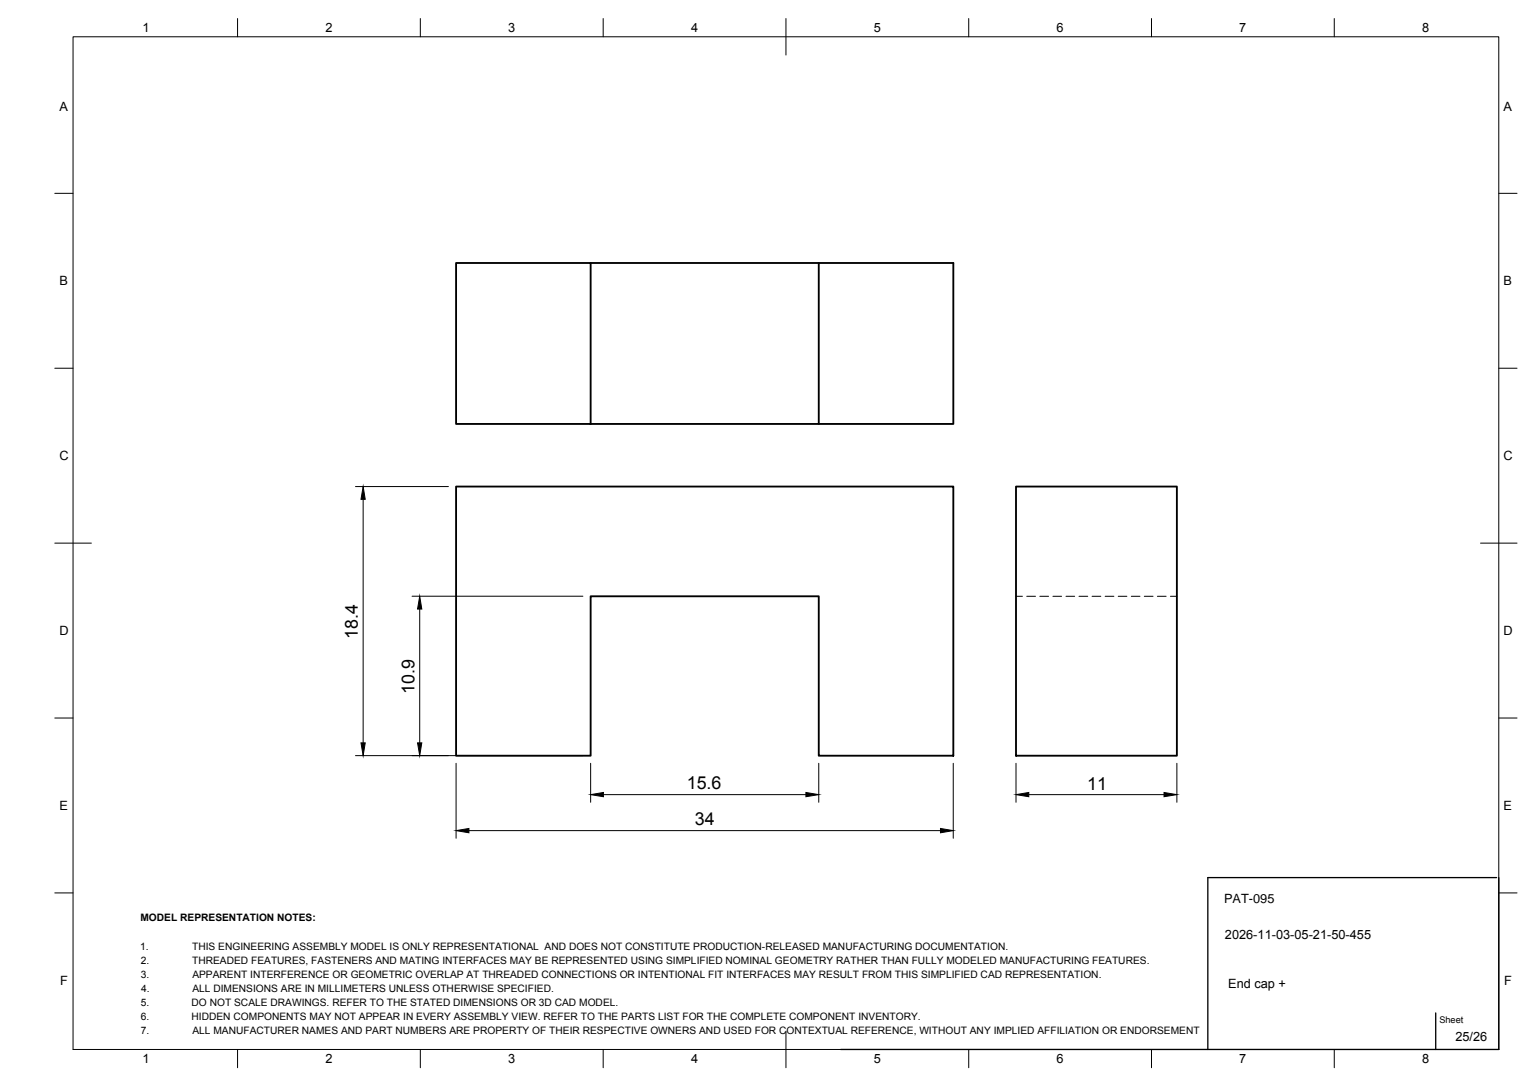
ISO-10303-21;
HEADER;
/* Generated by software containing ST-Developer
 * from STEP Tools, Inc. (www.steptools.com) 
 */

FILE_DESCRIPTION(
/* description */ ('Single-Axis Profile-Rail Linear Slide'),
/* implementation_level */ '2;1');

FILE_NAME(
/* name */ 'End cap +.step',
/* time_stamp */ '2026-10-27T10:47:43-07:00',
/* author */ (''),
/* organization */ (''),
/* preprocessor_version */ 'ST-DEVELOPER v20.2',
/* originating_system */ 'Autodesk Translation Framework v15.17.0.0',
/* authorisation */ '');

FILE_SCHEMA (('AUTOMOTIVE_DESIGN { 1 0 10303 214 3 1 1 }'));
ENDSEC;

DATA;
#10=MECHANICAL_DESIGN_GEOMETRIC_PRESENTATION_REPRESENTATION('',(#348),#14478);
#294=SHAPE_REPRESENTATION_RELATIONSHIP('SRR','None',#14626,#321);
#321=ADVANCED_BREP_SHAPE_REPRESENTATION('',(#373),#14470);
#348=STYLED_ITEM('',(#14824),#373);
#373=MANIFOLD_SOLID_BREP('Body1',#8610);
#781=PLANE('',#9433);
#782=PLANE('',#9434);
#783=PLANE('',#9435);
#784=PLANE('',#9436);
#785=PLANE('',#9437);
#786=PLANE('',#9438);
#787=PLANE('',#9439);
#788=PLANE('',#9440);
#789=PLANE('',#9441);
#790=PLANE('',#9442);
#1210=FACE_OUTER_BOUND('',#1746,.T.);
#1211=FACE_OUTER_BOUND('',#1747,.T.);
#1212=FACE_OUTER_BOUND('',#1748,.T.);
#1213=FACE_OUTER_BOUND('',#1749,.T.);
#1214=FACE_OUTER_BOUND('',#1750,.T.);
#1215=FACE_OUTER_BOUND('',#1751,.T.);
#1216=FACE_OUTER_BOUND('',#1752,.T.);
#1217=FACE_OUTER_BOUND('',#1753,.T.);
#1218=FACE_OUTER_BOUND('',#1754,.T.);
#1219=FACE_OUTER_BOUND('',#1755,.T.);
#1746=EDGE_LOOP('',(#7739,#7740,#7741,#7742));
#1747=EDGE_LOOP('',(#7743,#7744,#7745,#7746));
#1748=EDGE_LOOP('',(#7747,#7748,#7749,#7750));
#1749=EDGE_LOOP('',(#7751,#7752,#7753,#7754));
#1750=EDGE_LOOP('',(#7755,#7756,#7757,#7758));
#1751=EDGE_LOOP('',(#7759,#7760,#7761,#7762));
#1752=EDGE_LOOP('',(#7763,#7764,#7765,#7766));
#1753=EDGE_LOOP('',(#7767,#7768,#7769,#7770));
#1754=EDGE_LOOP('',(#7771,#7772,#7773,#7774,#7775,#7776,#7777,#7778));
#1755=EDGE_LOOP('',(#7779,#7780,#7781,#7782,#7783,#7784,#7785,#7786));
#2683=LINE('',#13996,#3654);
#2684=LINE('',#13998,#3655);
#2685=LINE('',#14000,#3656);
#2686=LINE('',#14001,#3657);
#2687=LINE('',#14004,#3658);
#2688=LINE('',#14006,#3659);
#2689=LINE('',#14007,#3660);
#2690=LINE('',#14010,#3661);
#2691=LINE('',#14012,#3662);
#2692=LINE('',#14013,#3663);
#2693=LINE('',#14016,#3664);
#2694=LINE('',#14018,#3665);
#2695=LINE('',#14019,#3666);
#2696=LINE('',#14022,#3667);
#2697=LINE('',#14024,#3668);
#2698=LINE('',#14025,#3669);
#2699=LINE('',#14028,#3670);
#2700=LINE('',#14030,#3671);
#2701=LINE('',#14031,#3672);
#2702=LINE('',#14034,#3673);
#2703=LINE('',#14036,#3674);
#2704=LINE('',#14037,#3675);
#2705=LINE('',#14039,#3676);
#2706=LINE('',#14040,#3677);
#3654=VECTOR('',#11494,1.);
#3655=VECTOR('',#11495,1.);
#3656=VECTOR('',#11496,1.);
#3657=VECTOR('',#11497,1.);
#3658=VECTOR('',#11500,1.);
#3659=VECTOR('',#11501,1.);
#3660=VECTOR('',#11502,1.);
#3661=VECTOR('',#11505,1.);
#3662=VECTOR('',#11506,1.);
#3663=VECTOR('',#11507,1.);
#3664=VECTOR('',#11510,1.);
#3665=VECTOR('',#11511,1.);
#3666=VECTOR('',#11512,1.);
#3667=VECTOR('',#11515,1.);
#3668=VECTOR('',#11516,1.);
#3669=VECTOR('',#11517,1.);
#3670=VECTOR('',#11520,1.);
#3671=VECTOR('',#11521,1.);
#3672=VECTOR('',#11522,1.);
#3673=VECTOR('',#11525,1.);
#3674=VECTOR('',#11526,1.);
#3675=VECTOR('',#11527,1.);
#3676=VECTOR('',#11530,1.);
#3677=VECTOR('',#11531,1.);
#4578=VERTEX_POINT('',#13994);
#4579=VERTEX_POINT('',#13995);
#4580=VERTEX_POINT('',#13997);
#4581=VERTEX_POINT('',#13999);
#4582=VERTEX_POINT('',#14003);
#4583=VERTEX_POINT('',#14005);
#4584=VERTEX_POINT('',#14009);
#4585=VERTEX_POINT('',#14011);
#4586=VERTEX_POINT('',#14015);
#4587=VERTEX_POINT('',#14017);
#4588=VERTEX_POINT('',#14021);
#4589=VERTEX_POINT('',#14023);
#4590=VERTEX_POINT('',#14027);
#4591=VERTEX_POINT('',#14029);
#4592=VERTEX_POINT('',#14033);
#4593=VERTEX_POINT('',#14035);
#5647=EDGE_CURVE('',#4578,#4579,#2683,.T.);
#5648=EDGE_CURVE('',#4579,#4580,#2684,.T.);
#5649=EDGE_CURVE('',#4581,#4580,#2685,.T.);
#5650=EDGE_CURVE('',#4578,#4581,#2686,.T.);
#5651=EDGE_CURVE('',#4582,#4578,#2687,.T.);
#5652=EDGE_CURVE('',#4583,#4581,#2688,.T.);
#5653=EDGE_CURVE('',#4582,#4583,#2689,.T.);
#5654=EDGE_CURVE('',#4584,#4582,#2690,.T.);
#5655=EDGE_CURVE('',#4585,#4583,#2691,.T.);
#5656=EDGE_CURVE('',#4584,#4585,#2692,.T.);
#5657=EDGE_CURVE('',#4586,#4584,#2693,.T.);
#5658=EDGE_CURVE('',#4587,#4585,#2694,.T.);
#5659=EDGE_CURVE('',#4586,#4587,#2695,.T.);
#5660=EDGE_CURVE('',#4588,#4586,#2696,.T.);
#5661=EDGE_CURVE('',#4589,#4587,#2697,.T.);
#5662=EDGE_CURVE('',#4588,#4589,#2698,.T.);
#5663=EDGE_CURVE('',#4590,#4588,#2699,.T.);
#5664=EDGE_CURVE('',#4591,#4589,#2700,.T.);
#5665=EDGE_CURVE('',#4590,#4591,#2701,.T.);
#5666=EDGE_CURVE('',#4592,#4590,#2702,.T.);
#5667=EDGE_CURVE('',#4593,#4591,#2703,.T.);
#5668=EDGE_CURVE('',#4592,#4593,#2704,.T.);
#5669=EDGE_CURVE('',#4579,#4592,#2705,.T.);
#5670=EDGE_CURVE('',#4580,#4593,#2706,.T.);
#7739=ORIENTED_EDGE('',*,*,#5647,.T.);
#7740=ORIENTED_EDGE('',*,*,#5648,.T.);
#7741=ORIENTED_EDGE('',*,*,#5649,.F.);
#7742=ORIENTED_EDGE('',*,*,#5650,.F.);
#7743=ORIENTED_EDGE('',*,*,#5651,.T.);
#7744=ORIENTED_EDGE('',*,*,#5650,.T.);
#7745=ORIENTED_EDGE('',*,*,#5652,.F.);
#7746=ORIENTED_EDGE('',*,*,#5653,.F.);
#7747=ORIENTED_EDGE('',*,*,#5654,.T.);
#7748=ORIENTED_EDGE('',*,*,#5653,.T.);
#7749=ORIENTED_EDGE('',*,*,#5655,.F.);
#7750=ORIENTED_EDGE('',*,*,#5656,.F.);
#7751=ORIENTED_EDGE('',*,*,#5657,.T.);
#7752=ORIENTED_EDGE('',*,*,#5656,.T.);
#7753=ORIENTED_EDGE('',*,*,#5658,.F.);
#7754=ORIENTED_EDGE('',*,*,#5659,.F.);
#7755=ORIENTED_EDGE('',*,*,#5660,.T.);
#7756=ORIENTED_EDGE('',*,*,#5659,.T.);
#7757=ORIENTED_EDGE('',*,*,#5661,.F.);
#7758=ORIENTED_EDGE('',*,*,#5662,.F.);
#7759=ORIENTED_EDGE('',*,*,#5663,.T.);
#7760=ORIENTED_EDGE('',*,*,#5662,.T.);
#7761=ORIENTED_EDGE('',*,*,#5664,.F.);
#7762=ORIENTED_EDGE('',*,*,#5665,.F.);
#7763=ORIENTED_EDGE('',*,*,#5666,.T.);
#7764=ORIENTED_EDGE('',*,*,#5665,.T.);
#7765=ORIENTED_EDGE('',*,*,#5667,.F.);
#7766=ORIENTED_EDGE('',*,*,#5668,.F.);
#7767=ORIENTED_EDGE('',*,*,#5669,.T.);
#7768=ORIENTED_EDGE('',*,*,#5668,.T.);
#7769=ORIENTED_EDGE('',*,*,#5670,.F.);
#7770=ORIENTED_EDGE('',*,*,#5648,.F.);
#7771=ORIENTED_EDGE('',*,*,#5670,.T.);
#7772=ORIENTED_EDGE('',*,*,#5667,.T.);
#7773=ORIENTED_EDGE('',*,*,#5664,.T.);
#7774=ORIENTED_EDGE('',*,*,#5661,.T.);
#7775=ORIENTED_EDGE('',*,*,#5658,.T.);
#7776=ORIENTED_EDGE('',*,*,#5655,.T.);
#7777=ORIENTED_EDGE('',*,*,#5652,.T.);
#7778=ORIENTED_EDGE('',*,*,#5649,.T.);
#7779=ORIENTED_EDGE('',*,*,#5669,.F.);
#7780=ORIENTED_EDGE('',*,*,#5647,.F.);
#7781=ORIENTED_EDGE('',*,*,#5651,.F.);
#7782=ORIENTED_EDGE('',*,*,#5654,.F.);
#7783=ORIENTED_EDGE('',*,*,#5657,.F.);
#7784=ORIENTED_EDGE('',*,*,#5660,.F.);
#7785=ORIENTED_EDGE('',*,*,#5663,.F.);
#7786=ORIENTED_EDGE('',*,*,#5666,.F.);
#8504=ADVANCED_FACE('',(#1210),#781,.T.);
#8505=ADVANCED_FACE('',(#1211),#782,.T.);
#8506=ADVANCED_FACE('',(#1212),#783,.T.);
#8507=ADVANCED_FACE('',(#1213),#784,.T.);
#8508=ADVANCED_FACE('',(#1214),#785,.T.);
#8509=ADVANCED_FACE('',(#1215),#786,.T.);
#8510=ADVANCED_FACE('',(#1216),#787,.T.);
#8511=ADVANCED_FACE('',(#1217),#788,.T.);
#8512=ADVANCED_FACE('',(#1218),#789,.T.);
#8513=ADVANCED_FACE('',(#1219),#790,.F.);
#8610=CLOSED_SHELL('',(#8504,#8505,#8506,#8507,#8508,#8509,#8510,#8511,
#8512,#8513));
#9432=AXIS2_PLACEMENT_3D('',#13992,#11490,#11491);
#9433=AXIS2_PLACEMENT_3D('',#13993,#11492,#11493);
#9434=AXIS2_PLACEMENT_3D('',#14002,#11498,#11499);
#9435=AXIS2_PLACEMENT_3D('',#14008,#11503,#11504);
#9436=AXIS2_PLACEMENT_3D('',#14014,#11508,#11509);
#9437=AXIS2_PLACEMENT_3D('',#14020,#11513,#11514);
#9438=AXIS2_PLACEMENT_3D('',#14026,#11518,#11519);
#9439=AXIS2_PLACEMENT_3D('',#14032,#11523,#11524);
#9440=AXIS2_PLACEMENT_3D('',#14038,#11528,#11529);
#9441=AXIS2_PLACEMENT_3D('',#14041,#11532,#11533);
#9442=AXIS2_PLACEMENT_3D('',#14042,#11534,#11535);
#11490=DIRECTION('axis',(0.,0.,1.));
#11491=DIRECTION('refdir',(1.,0.,0.));
#11492=DIRECTION('center_axis',(0.,0.,1.));
#11493=DIRECTION('ref_axis',(0.,-1.,0.));
#11494=DIRECTION('',(0.,-1.,0.));
#11495=DIRECTION('',(1.,0.,0.));
#11496=DIRECTION('',(0.,-1.,0.));
#11497=DIRECTION('',(1.,0.,0.));
#11498=DIRECTION('center_axis',(0.,1.,0.));
#11499=DIRECTION('ref_axis',(0.,0.,1.));
#11500=DIRECTION('',(0.,0.,1.));
#11501=DIRECTION('',(0.,0.,1.));
#11502=DIRECTION('',(1.,0.,0.));
#11503=DIRECTION('center_axis',(0.,0.,-1.));
#11504=DIRECTION('ref_axis',(0.,1.,0.));
#11505=DIRECTION('',(0.,1.,0.));
#11506=DIRECTION('',(0.,1.,0.));
#11507=DIRECTION('',(1.,0.,0.));
#11508=DIRECTION('center_axis',(0.,-1.,0.));
#11509=DIRECTION('ref_axis',(0.,0.,-1.));
#11510=DIRECTION('',(0.,0.,-1.));
#11511=DIRECTION('',(0.,0.,-1.));
#11512=DIRECTION('',(1.,0.,0.));
#11513=DIRECTION('center_axis',(0.,0.,-1.));
#11514=DIRECTION('ref_axis',(0.,1.,0.));
#11515=DIRECTION('',(0.,1.,0.));
#11516=DIRECTION('',(0.,1.,0.));
#11517=DIRECTION('',(1.,0.,0.));
#11518=DIRECTION('center_axis',(0.,1.,0.));
#11519=DIRECTION('ref_axis',(0.,0.,1.));
#11520=DIRECTION('',(0.,0.,1.));
#11521=DIRECTION('',(0.,0.,1.));
#11522=DIRECTION('',(1.,0.,0.));
#11523=DIRECTION('center_axis',(0.,0.,-1.));
#11524=DIRECTION('ref_axis',(0.,1.,0.));
#11525=DIRECTION('',(0.,1.,0.));
#11526=DIRECTION('',(0.,1.,0.));
#11527=DIRECTION('',(1.,0.,0.));
#11528=DIRECTION('center_axis',(0.,-1.,0.));
#11529=DIRECTION('ref_axis',(0.,0.,-1.));
#11530=DIRECTION('',(0.,0.,-1.));
#11531=DIRECTION('',(0.,0.,-1.));
#11532=DIRECTION('center_axis',(1.,0.,0.));
#11533=DIRECTION('ref_axis',(0.,0.,-1.));
#11534=DIRECTION('center_axis',(1.,0.,0.));
#11535=DIRECTION('ref_axis',(0.,0.,-1.));
#13992=CARTESIAN_POINT('',(0.,0.,0.));
#13993=CARTESIAN_POINT('Origin',(1.97,1.7,2.3));
#13994=CARTESIAN_POINT('',(1.97,1.7,2.3));
#13995=CARTESIAN_POINT('',(1.97,-1.7,2.3));
#13996=CARTESIAN_POINT('',(1.97,1.7,2.3));
#13997=CARTESIAN_POINT('',(3.07,-1.7,2.3));
#13998=CARTESIAN_POINT('',(1.97,-1.7,2.3));
#13999=CARTESIAN_POINT('',(3.07,1.7,2.3));
#14000=CARTESIAN_POINT('',(3.07,1.7,2.3));
#14001=CARTESIAN_POINT('',(1.97,1.7,2.3));
#14002=CARTESIAN_POINT('Origin',(1.97,1.7,0.46));
#14003=CARTESIAN_POINT('',(1.97,1.7,0.46));
#14004=CARTESIAN_POINT('',(1.97,1.7,0.46));
#14005=CARTESIAN_POINT('',(3.07,1.7,0.46));
#14006=CARTESIAN_POINT('',(3.07,1.7,0.46));
#14007=CARTESIAN_POINT('',(1.97,1.7,0.46));
#14008=CARTESIAN_POINT('Origin',(1.97,0.78,0.46));
#14009=CARTESIAN_POINT('',(1.97,0.78,0.46));
#14010=CARTESIAN_POINT('',(1.97,0.78,0.46));
#14011=CARTESIAN_POINT('',(3.07,0.78,0.46));
#14012=CARTESIAN_POINT('',(3.07,0.78,0.46));
#14013=CARTESIAN_POINT('',(1.97,0.78,0.46));
#14014=CARTESIAN_POINT('Origin',(1.97,0.78,1.55));
#14015=CARTESIAN_POINT('',(1.97,0.78,1.55));
#14016=CARTESIAN_POINT('',(1.97,0.78,1.55));
#14017=CARTESIAN_POINT('',(3.07,0.78,1.55));
#14018=CARTESIAN_POINT('',(3.07,0.78,1.55));
#14019=CARTESIAN_POINT('',(1.97,0.78,1.55));
#14020=CARTESIAN_POINT('Origin',(1.97,-0.78,1.55));
#14021=CARTESIAN_POINT('',(1.97,-0.78,1.55));
#14022=CARTESIAN_POINT('',(1.97,-0.78,1.55));
#14023=CARTESIAN_POINT('',(3.07,-0.78,1.55));
#14024=CARTESIAN_POINT('',(3.07,-0.78,1.55));
#14025=CARTESIAN_POINT('',(1.97,-0.78,1.55));
#14026=CARTESIAN_POINT('Origin',(1.97,-0.78,0.46));
#14027=CARTESIAN_POINT('',(1.97,-0.78,0.46));
#14028=CARTESIAN_POINT('',(1.97,-0.78,0.46));
#14029=CARTESIAN_POINT('',(3.07,-0.78,0.46));
#14030=CARTESIAN_POINT('',(3.07,-0.78,0.46));
#14031=CARTESIAN_POINT('',(1.97,-0.78,0.46));
#14032=CARTESIAN_POINT('Origin',(1.97,-1.7,0.46));
#14033=CARTESIAN_POINT('',(1.97,-1.7,0.46));
#14034=CARTESIAN_POINT('',(1.97,-1.7,0.46));
#14035=CARTESIAN_POINT('',(3.07,-1.7,0.46));
#14036=CARTESIAN_POINT('',(3.07,-1.7,0.46));
#14037=CARTESIAN_POINT('',(1.97,-1.7,0.46));
#14038=CARTESIAN_POINT('Origin',(1.97,-1.7,2.3));
#14039=CARTESIAN_POINT('',(1.97,-1.7,2.3));
#14040=CARTESIAN_POINT('',(3.07,-1.7,2.3));
#14041=CARTESIAN_POINT('Origin',(3.07,0.,1.38));
#14042=CARTESIAN_POINT('Origin',(1.97,0.,1.38));
#14438=UNCERTAINTY_MEASURE_WITH_UNIT(LENGTH_MEASURE(0.001),#14479,
'DISTANCE_ACCURACY_VALUE',
'Maximum model space distance between geometric entities at asserted c
onnectivities');
#14446=UNCERTAINTY_MEASURE_WITH_UNIT(LENGTH_MEASURE(0.001),#14479,
'DISTANCE_ACCURACY_VALUE',
'Maximum model space distance between geometric entities at asserted c
onnectivities');
#14470=(
GEOMETRIC_REPRESENTATION_CONTEXT(3)
GLOBAL_UNCERTAINTY_ASSIGNED_CONTEXT((#14438))
GLOBAL_UNIT_ASSIGNED_CONTEXT((#14479,#14481,#14482))
REPRESENTATION_CONTEXT('','3D')
);
#14478=(
GEOMETRIC_REPRESENTATION_CONTEXT(3)
GLOBAL_UNCERTAINTY_ASSIGNED_CONTEXT((#14446))
GLOBAL_UNIT_ASSIGNED_CONTEXT((#14479,#14481,#14482))
REPRESENTATION_CONTEXT('','3D')
);
#14479=(
LENGTH_UNIT()
NAMED_UNIT(*)
SI_UNIT(.CENTI.,.METRE.)
);
#14481=(
NAMED_UNIT(*)
PLANE_ANGLE_UNIT()
SI_UNIT($,.RADIAN.)
);
#14482=(
NAMED_UNIT(*)
SI_UNIT($,.STERADIAN.)
SOLID_ANGLE_UNIT()
);
#14506=SHAPE_DEFINITION_REPRESENTATION(#14537,#14626);
#14537=PRODUCT_DEFINITION_SHAPE('',$,#14658);
#14626=SHAPE_REPRESENTATION('',(#9432),#14470);
#14634=PRODUCT_DEFINITION_CONTEXT('part definition',#14729,'design');
#14658=PRODUCT_DEFINITION('End cap +','End cap +',#14689,#14634);
#14689=PRODUCT_DEFINITION_FORMATION('',$,#14754);
#14729=APPLICATION_CONTEXT(
'Core Data for Automotive Mechanical Design Process');
#14730=PRODUCT_CONTEXT('part definition',#14729,'mechanical');
#14754=PRODUCT('End cap +','End cap +','End cap +',(#14730));
#14818=COLOUR_RGB('Sky Blue',0.24,0.69,0.87);
#14819=FILL_AREA_STYLE_COLOUR('',#14818);
#14820=FILL_AREA_STYLE('',(#14819));
#14821=SURFACE_STYLE_FILL_AREA(#14820);
#14822=SURFACE_SIDE_STYLE('',(#14821));
#14823=SURFACE_STYLE_USAGE(.BOTH.,#14822);
#14824=PRESENTATION_STYLE_ASSIGNMENT((#14823));
ENDSEC;
END-ISO-10303-21;
